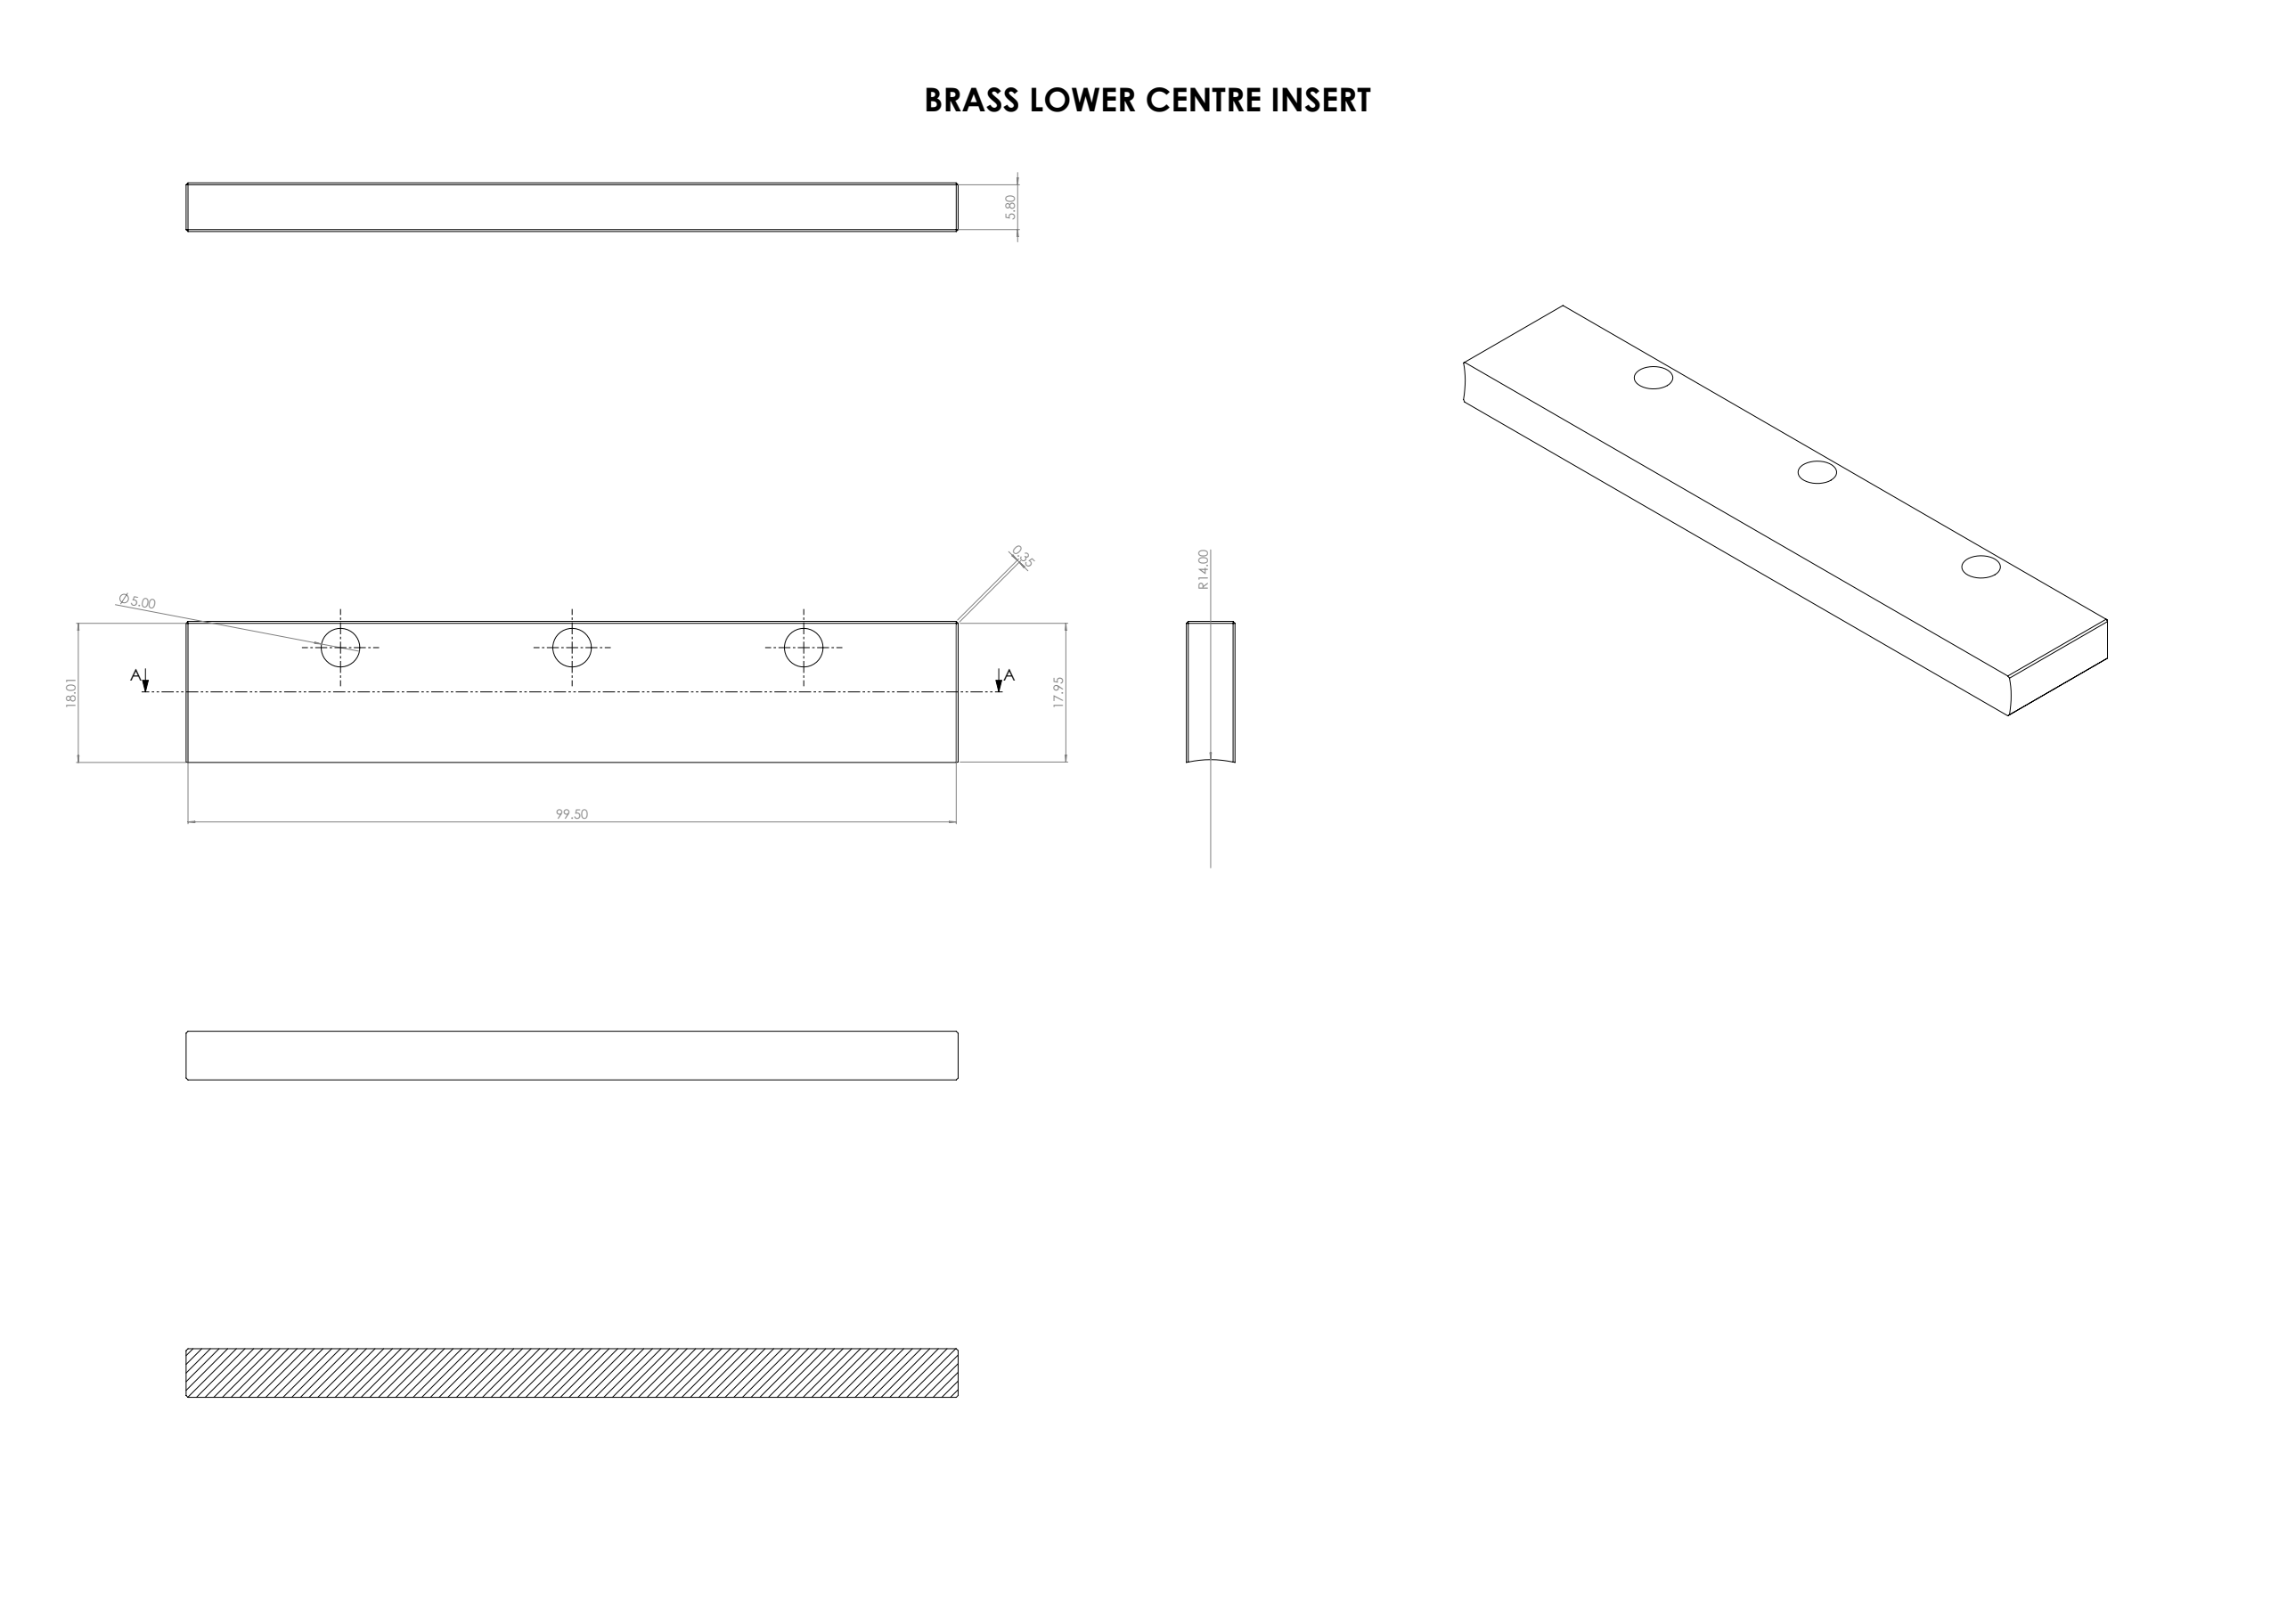
ISO-10303-21;
HEADER;
/* Generated by software containing ST-Developer
 * from STEP Tools, Inc. (www.steptools.com) 
 */

FILE_DESCRIPTION(
/* description */ (''),
/* implementation_level */ '2;1');

FILE_NAME(
/* name */ '02_Brass_Lower_Centre_Insert.step',
/* time_stamp */ '2026-10-21T01:59:45-07:00',
/* author */ (''),
/* organization */ (''),
/* preprocessor_version */ 'ST-DEVELOPER v20.2',
/* originating_system */ 'Autodesk Translation Framework v15.15.0.0',
/* authorisation */ '');

FILE_SCHEMA (('AUTOMOTIVE_DESIGN { 1 0 10303 214 3 1 1 }'));
ENDSEC;

DATA;
#10=MECHANICAL_DESIGN_GEOMETRIC_PRESENTATION_REPRESENTATION('',(#463),#18281);
#437=SHAPE_REPRESENTATION_RELATIONSHIP('SRR','None',#18339,#450);
#450=ADVANCED_BREP_SHAPE_REPRESENTATION('',(#481),#18268);
#463=STYLED_ITEM('',(#18467),#481);
#481=MANIFOLD_SOLID_BREP('Body1',#9085);
#494=CYLINDRICAL_SURFACE('',#9267,2.5);
#495=CYLINDRICAL_SURFACE('',#9269,2.5);
#496=CYLINDRICAL_SURFACE('',#9271,2.5);
#497=CYLINDRICAL_SURFACE('',#9273,14.);
#579=FACE_BOUND('',#1377,.T.);
#580=FACE_BOUND('',#1378,.T.);
#581=FACE_BOUND('',#1379,.T.);
#582=FACE_BOUND('',#1388,.T.);
#583=FACE_BOUND('',#1389,.T.);
#584=FACE_BOUND('',#1390,.T.);
#629=CIRCLE('',#9261,2.5);
#630=CIRCLE('',#9262,2.5);
#631=CIRCLE('',#9263,2.5);
#632=CIRCLE('',#9265,14.);
#633=CIRCLE('',#9268,2.5);
#634=CIRCLE('',#9270,2.5);
#635=CIRCLE('',#9272,2.5);
#636=CIRCLE('',#9274,14.);
#822=ELLIPSE('',#9249,19.7989898732233,14.);
#823=ELLIPSE('',#9254,19.7989898732235,14.);
#824=ELLIPSE('',#9256,19.7989898732233,14.);
#825=ELLIPSE('',#9259,19.7989898732235,14.);
#842=FACE_OUTER_BOUND('',#1364,.T.);
#843=FACE_OUTER_BOUND('',#1365,.T.);
#844=FACE_OUTER_BOUND('',#1366,.T.);
#845=FACE_OUTER_BOUND('',#1367,.T.);
#846=FACE_OUTER_BOUND('',#1368,.T.);
#847=FACE_OUTER_BOUND('',#1369,.T.);
#848=FACE_OUTER_BOUND('',#1370,.T.);
#849=FACE_OUTER_BOUND('',#1371,.T.);
#850=FACE_OUTER_BOUND('',#1372,.T.);
#851=FACE_OUTER_BOUND('',#1373,.T.);
#852=FACE_OUTER_BOUND('',#1374,.T.);
#853=FACE_OUTER_BOUND('',#1375,.T.);
#854=FACE_OUTER_BOUND('',#1376,.T.);
#855=FACE_OUTER_BOUND('',#1380,.T.);
#856=FACE_OUTER_BOUND('',#1381,.T.);
#857=FACE_OUTER_BOUND('',#1382,.T.);
#858=FACE_OUTER_BOUND('',#1383,.T.);
#859=FACE_OUTER_BOUND('',#1384,.T.);
#860=FACE_OUTER_BOUND('',#1385,.T.);
#861=FACE_OUTER_BOUND('',#1386,.T.);
#862=FACE_OUTER_BOUND('',#1387,.T.);
#1364=EDGE_LOOP('',(#5692,#5693,#5694));
#1365=EDGE_LOOP('',(#5695,#5696,#5697));
#1366=EDGE_LOOP('',(#5698,#5699,#5700));
#1367=EDGE_LOOP('',(#5701,#5702,#5703));
#1368=EDGE_LOOP('',(#5704,#5705,#5706,#5707));
#1369=EDGE_LOOP('',(#5708,#5709,#5710,#5711));
#1370=EDGE_LOOP('',(#5712,#5713,#5714,#5715));
#1371=EDGE_LOOP('',(#5716,#5717,#5718,#5719));
#1372=EDGE_LOOP('',(#5720,#5721,#5722,#5723));
#1373=EDGE_LOOP('',(#5724,#5725,#5726,#5727));
#1374=EDGE_LOOP('',(#5728,#5729,#5730,#5731));
#1375=EDGE_LOOP('',(#5732,#5733,#5734,#5735));
#1376=EDGE_LOOP('',(#5736,#5737,#5738,#5739));
#1377=EDGE_LOOP('',(#5740));
#1378=EDGE_LOOP('',(#5741));
#1379=EDGE_LOOP('',(#5742));
#1380=EDGE_LOOP('',(#5743,#5744,#5745,#5746));
#1381=EDGE_LOOP('',(#5747,#5748,#5749,#5750));
#1382=EDGE_LOOP('',(#5751,#5752,#5753,#5754));
#1383=EDGE_LOOP('',(#5755,#5756,#5757,#5758));
#1384=EDGE_LOOP('',(#5759,#5760,#5761,#5762));
#1385=EDGE_LOOP('',(#5763,#5764,#5765,#5766,#5767,#5768,#5769,#5770));
#1386=EDGE_LOOP('',(#5771,#5772,#5773,#5774));
#1387=EDGE_LOOP('',(#5775,#5776,#5777,#5778));
#1388=EDGE_LOOP('',(#5779));
#1389=EDGE_LOOP('',(#5780));
#1390=EDGE_LOOP('',(#5781));
#1936=LINE('',#12276,#2781);
#1937=LINE('',#12278,#2782);
#1938=LINE('',#12279,#2783);
#1939=LINE('',#12283,#2784);
#1940=LINE('',#12285,#2785);
#1941=LINE('',#12286,#2786);
#1942=LINE('',#12290,#2787);
#1943=LINE('',#12292,#2788);
#1944=LINE('',#12293,#2789);
#1945=LINE('',#12297,#2790);
#1946=LINE('',#12299,#2791);
#1947=LINE('',#12300,#2792);
#1948=LINE('',#12305,#2793);
#1949=LINE('',#12306,#2794);
#1950=LINE('',#12308,#2795);
#1951=LINE('',#12309,#2796);
#1952=LINE('',#12311,#2797);
#1953=LINE('',#12312,#2798);
#1954=LINE('',#12314,#2799);
#1955=LINE('',#12315,#2800);
#1956=LINE('',#12320,#2801);
#1957=LINE('',#12321,#2802);
#1958=LINE('',#12326,#2803);
#1959=LINE('',#12327,#2804);
#1960=LINE('',#12329,#2805);
#1961=LINE('',#12330,#2806);
#1962=LINE('',#12335,#2807);
#1963=LINE('',#12336,#2808);
#1964=LINE('',#12338,#2809);
#1965=LINE('',#12351,#2810);
#1966=LINE('',#12355,#2811);
#1967=LINE('',#12359,#2812);
#1968=LINE('',#12361,#2813);
#2781=VECTOR('',#9976,10.);
#2782=VECTOR('',#9977,10.);
#2783=VECTOR('',#9978,10.);
#2784=VECTOR('',#9981,10.);
#2785=VECTOR('',#9982,10.);
#2786=VECTOR('',#9983,10.);
#2787=VECTOR('',#9986,10.);
#2788=VECTOR('',#9987,10.);
#2789=VECTOR('',#9988,10.);
#2790=VECTOR('',#9991,10.);
#2791=VECTOR('',#9992,10.);
#2792=VECTOR('',#9993,10.);
#2793=VECTOR('',#9998,10.);
#2794=VECTOR('',#9999,10.);
#2795=VECTOR('',#10002,10.);
#2796=VECTOR('',#10003,10.);
#2797=VECTOR('',#10006,10.);
#2798=VECTOR('',#10007,10.);
#2799=VECTOR('',#10010,10.);
#2800=VECTOR('',#10011,10.);
#2801=VECTOR('',#10016,10.);
#2802=VECTOR('',#10017,10.);
#2803=VECTOR('',#10022,10.);
#2804=VECTOR('',#10023,10.);
#2805=VECTOR('',#10026,10.);
#2806=VECTOR('',#10027,10.);
#2807=VECTOR('',#10032,10.);
#2808=VECTOR('',#10033,10.);
#2809=VECTOR('',#10036,10.);
#2810=VECTOR('',#10053,2.5);
#2811=VECTOR('',#10058,2.5);
#2812=VECTOR('',#10063,2.5);
#2813=VECTOR('',#10066,10.);
#3626=VERTEX_POINT('',#12274);
#3627=VERTEX_POINT('',#12275);
#3628=VERTEX_POINT('',#12277);
#3629=VERTEX_POINT('',#12281);
#3630=VERTEX_POINT('',#12282);
#3631=VERTEX_POINT('',#12284);
#3632=VERTEX_POINT('',#12288);
#3633=VERTEX_POINT('',#12289);
#3634=VERTEX_POINT('',#12291);
#3635=VERTEX_POINT('',#12295);
#3636=VERTEX_POINT('',#12296);
#3637=VERTEX_POINT('',#12298);
#3638=VERTEX_POINT('',#12302);
#3639=VERTEX_POINT('',#12303);
#3640=VERTEX_POINT('',#12317);
#3641=VERTEX_POINT('',#12318);
#3642=VERTEX_POINT('',#12323);
#3643=VERTEX_POINT('',#12324);
#3644=VERTEX_POINT('',#12332);
#3645=VERTEX_POINT('',#12333);
#3646=VERTEX_POINT('',#12339);
#3647=VERTEX_POINT('',#12341);
#3648=VERTEX_POINT('',#12343);
#3649=VERTEX_POINT('',#12349);
#3650=VERTEX_POINT('',#12353);
#3651=VERTEX_POINT('',#12357);
#4418=EDGE_CURVE('',#3626,#3627,#1936,.T.);
#4419=EDGE_CURVE('',#3628,#3626,#1937,.T.);
#4420=EDGE_CURVE('',#3627,#3628,#1938,.T.);
#4421=EDGE_CURVE('',#3629,#3630,#1939,.T.);
#4422=EDGE_CURVE('',#3631,#3629,#1940,.T.);
#4423=EDGE_CURVE('',#3630,#3631,#1941,.T.);
#4424=EDGE_CURVE('',#3632,#3633,#1942,.T.);
#4425=EDGE_CURVE('',#3634,#3632,#1943,.T.);
#4426=EDGE_CURVE('',#3633,#3634,#1944,.T.);
#4427=EDGE_CURVE('',#3635,#3636,#1945,.T.);
#4428=EDGE_CURVE('',#3637,#3635,#1946,.T.);
#4429=EDGE_CURVE('',#3636,#3637,#1947,.T.);
#4430=EDGE_CURVE('',#3638,#3639,#822,.T.);
#4431=EDGE_CURVE('',#3639,#3637,#1948,.T.);
#4432=EDGE_CURVE('',#3635,#3638,#1949,.T.);
#4433=EDGE_CURVE('',#3629,#3636,#1950,.T.);
#4434=EDGE_CURVE('',#3637,#3631,#1951,.T.);
#4435=EDGE_CURVE('',#3632,#3635,#1952,.T.);
#4436=EDGE_CURVE('',#3636,#3634,#1953,.T.);
#4437=EDGE_CURVE('',#3627,#3633,#1954,.T.);
#4438=EDGE_CURVE('',#3634,#3626,#1955,.T.);
#4439=EDGE_CURVE('',#3640,#3641,#823,.T.);
#4440=EDGE_CURVE('',#3641,#3632,#1956,.T.);
#4441=EDGE_CURVE('',#3633,#3640,#1957,.T.);
#4442=EDGE_CURVE('',#3642,#3643,#824,.T.);
#4443=EDGE_CURVE('',#3643,#3630,#1958,.T.);
#4444=EDGE_CURVE('',#3631,#3642,#1959,.T.);
#4445=EDGE_CURVE('',#3626,#3629,#1960,.T.);
#4446=EDGE_CURVE('',#3630,#3628,#1961,.T.);
#4447=EDGE_CURVE('',#3644,#3645,#825,.T.);
#4448=EDGE_CURVE('',#3645,#3627,#1962,.T.);
#4449=EDGE_CURVE('',#3628,#3644,#1963,.T.);
#4450=EDGE_CURVE('',#3641,#3638,#1964,.T.);
#4451=EDGE_CURVE('',#3646,#3646,#629,.T.);
#4452=EDGE_CURVE('',#3647,#3647,#630,.T.);
#4453=EDGE_CURVE('',#3648,#3648,#631,.T.);
#4454=EDGE_CURVE('',#3645,#3640,#632,.T.);
#4455=EDGE_CURVE('',#3649,#3649,#633,.T.);
#4456=EDGE_CURVE('',#3649,#3648,#1965,.T.);
#4457=EDGE_CURVE('',#3650,#3650,#634,.T.);
#4458=EDGE_CURVE('',#3650,#3647,#1966,.T.);
#4459=EDGE_CURVE('',#3651,#3651,#635,.T.);
#4460=EDGE_CURVE('',#3651,#3646,#1967,.T.);
#4461=EDGE_CURVE('',#3643,#3644,#1968,.T.);
#4462=EDGE_CURVE('',#3639,#3642,#636,.T.);
#5692=ORIENTED_EDGE('',*,*,#4418,.F.);
#5693=ORIENTED_EDGE('',*,*,#4419,.F.);
#5694=ORIENTED_EDGE('',*,*,#4420,.F.);
#5695=ORIENTED_EDGE('',*,*,#4421,.F.);
#5696=ORIENTED_EDGE('',*,*,#4422,.F.);
#5697=ORIENTED_EDGE('',*,*,#4423,.F.);
#5698=ORIENTED_EDGE('',*,*,#4424,.F.);
#5699=ORIENTED_EDGE('',*,*,#4425,.F.);
#5700=ORIENTED_EDGE('',*,*,#4426,.F.);
#5701=ORIENTED_EDGE('',*,*,#4427,.F.);
#5702=ORIENTED_EDGE('',*,*,#4428,.F.);
#5703=ORIENTED_EDGE('',*,*,#4429,.F.);
#5704=ORIENTED_EDGE('',*,*,#4430,.T.);
#5705=ORIENTED_EDGE('',*,*,#4431,.T.);
#5706=ORIENTED_EDGE('',*,*,#4428,.T.);
#5707=ORIENTED_EDGE('',*,*,#4432,.T.);
#5708=ORIENTED_EDGE('',*,*,#4422,.T.);
#5709=ORIENTED_EDGE('',*,*,#4433,.T.);
#5710=ORIENTED_EDGE('',*,*,#4429,.T.);
#5711=ORIENTED_EDGE('',*,*,#4434,.T.);
#5712=ORIENTED_EDGE('',*,*,#4425,.T.);
#5713=ORIENTED_EDGE('',*,*,#4435,.T.);
#5714=ORIENTED_EDGE('',*,*,#4427,.T.);
#5715=ORIENTED_EDGE('',*,*,#4436,.T.);
#5716=ORIENTED_EDGE('',*,*,#4418,.T.);
#5717=ORIENTED_EDGE('',*,*,#4437,.T.);
#5718=ORIENTED_EDGE('',*,*,#4426,.T.);
#5719=ORIENTED_EDGE('',*,*,#4438,.T.);
#5720=ORIENTED_EDGE('',*,*,#4439,.T.);
#5721=ORIENTED_EDGE('',*,*,#4440,.T.);
#5722=ORIENTED_EDGE('',*,*,#4424,.T.);
#5723=ORIENTED_EDGE('',*,*,#4441,.T.);
#5724=ORIENTED_EDGE('',*,*,#4442,.T.);
#5725=ORIENTED_EDGE('',*,*,#4443,.T.);
#5726=ORIENTED_EDGE('',*,*,#4423,.T.);
#5727=ORIENTED_EDGE('',*,*,#4444,.T.);
#5728=ORIENTED_EDGE('',*,*,#4419,.T.);
#5729=ORIENTED_EDGE('',*,*,#4445,.T.);
#5730=ORIENTED_EDGE('',*,*,#4421,.T.);
#5731=ORIENTED_EDGE('',*,*,#4446,.T.);
#5732=ORIENTED_EDGE('',*,*,#4447,.T.);
#5733=ORIENTED_EDGE('',*,*,#4448,.T.);
#5734=ORIENTED_EDGE('',*,*,#4420,.T.);
#5735=ORIENTED_EDGE('',*,*,#4449,.T.);
#5736=ORIENTED_EDGE('',*,*,#4432,.F.);
#5737=ORIENTED_EDGE('',*,*,#4435,.F.);
#5738=ORIENTED_EDGE('',*,*,#4440,.F.);
#5739=ORIENTED_EDGE('',*,*,#4450,.T.);
#5740=ORIENTED_EDGE('',*,*,#4451,.T.);
#5741=ORIENTED_EDGE('',*,*,#4452,.T.);
#5742=ORIENTED_EDGE('',*,*,#4453,.T.);
#5743=ORIENTED_EDGE('',*,*,#4441,.F.);
#5744=ORIENTED_EDGE('',*,*,#4437,.F.);
#5745=ORIENTED_EDGE('',*,*,#4448,.F.);
#5746=ORIENTED_EDGE('',*,*,#4454,.T.);
#5747=ORIENTED_EDGE('',*,*,#4433,.F.);
#5748=ORIENTED_EDGE('',*,*,#4445,.F.);
#5749=ORIENTED_EDGE('',*,*,#4438,.F.);
#5750=ORIENTED_EDGE('',*,*,#4436,.F.);
#5751=ORIENTED_EDGE('',*,*,#4455,.F.);
#5752=ORIENTED_EDGE('',*,*,#4456,.T.);
#5753=ORIENTED_EDGE('',*,*,#4453,.F.);
#5754=ORIENTED_EDGE('',*,*,#4456,.F.);
#5755=ORIENTED_EDGE('',*,*,#4457,.F.);
#5756=ORIENTED_EDGE('',*,*,#4458,.T.);
#5757=ORIENTED_EDGE('',*,*,#4452,.F.);
#5758=ORIENTED_EDGE('',*,*,#4458,.F.);
#5759=ORIENTED_EDGE('',*,*,#4459,.F.);
#5760=ORIENTED_EDGE('',*,*,#4460,.T.);
#5761=ORIENTED_EDGE('',*,*,#4451,.F.);
#5762=ORIENTED_EDGE('',*,*,#4460,.F.);
#5763=ORIENTED_EDGE('',*,*,#4430,.F.);
#5764=ORIENTED_EDGE('',*,*,#4450,.F.);
#5765=ORIENTED_EDGE('',*,*,#4439,.F.);
#5766=ORIENTED_EDGE('',*,*,#4454,.F.);
#5767=ORIENTED_EDGE('',*,*,#4447,.F.);
#5768=ORIENTED_EDGE('',*,*,#4461,.F.);
#5769=ORIENTED_EDGE('',*,*,#4442,.F.);
#5770=ORIENTED_EDGE('',*,*,#4462,.F.);
#5771=ORIENTED_EDGE('',*,*,#4431,.F.);
#5772=ORIENTED_EDGE('',*,*,#4462,.T.);
#5773=ORIENTED_EDGE('',*,*,#4444,.F.);
#5774=ORIENTED_EDGE('',*,*,#4434,.F.);
#5775=ORIENTED_EDGE('',*,*,#4443,.F.);
#5776=ORIENTED_EDGE('',*,*,#4461,.T.);
#5777=ORIENTED_EDGE('',*,*,#4449,.F.);
#5778=ORIENTED_EDGE('',*,*,#4446,.F.);
#5779=ORIENTED_EDGE('',*,*,#4455,.T.);
#5780=ORIENTED_EDGE('',*,*,#4457,.T.);
#5781=ORIENTED_EDGE('',*,*,#4459,.T.);
#8240=PLANE('',#9244);
#8241=PLANE('',#9245);
#8242=PLANE('',#9246);
#8243=PLANE('',#9247);
#8244=PLANE('',#9248);
#8245=PLANE('',#9250);
#8246=PLANE('',#9251);
#8247=PLANE('',#9252);
#8248=PLANE('',#9253);
#8249=PLANE('',#9255);
#8250=PLANE('',#9257);
#8251=PLANE('',#9258);
#8252=PLANE('',#9260);
#8253=PLANE('',#9264);
#8254=PLANE('',#9266);
#8255=PLANE('',#9275);
#8256=PLANE('',#9276);
#8563=ADVANCED_FACE('',(#842),#8240,.T.);
#8564=ADVANCED_FACE('',(#843),#8241,.T.);
#8565=ADVANCED_FACE('',(#844),#8242,.T.);
#8566=ADVANCED_FACE('',(#845),#8243,.T.);
#8567=ADVANCED_FACE('',(#846),#8244,.T.);
#8568=ADVANCED_FACE('',(#847),#8245,.T.);
#8569=ADVANCED_FACE('',(#848),#8246,.T.);
#8570=ADVANCED_FACE('',(#849),#8247,.T.);
#8571=ADVANCED_FACE('',(#850),#8248,.T.);
#8572=ADVANCED_FACE('',(#851),#8249,.T.);
#8573=ADVANCED_FACE('',(#852),#8250,.T.);
#8574=ADVANCED_FACE('',(#853),#8251,.T.);
#8575=ADVANCED_FACE('',(#854,#579,#580,#581),#8252,.T.);
#8576=ADVANCED_FACE('',(#855),#8253,.T.);
#8577=ADVANCED_FACE('',(#856),#8254,.T.);
#8578=ADVANCED_FACE('',(#857),#494,.F.);
#8579=ADVANCED_FACE('',(#858),#495,.F.);
#8580=ADVANCED_FACE('',(#859),#496,.F.);
#8581=ADVANCED_FACE('',(#860),#497,.F.);
#8582=ADVANCED_FACE('',(#861),#8255,.F.);
#8583=ADVANCED_FACE('',(#862,#582,#583,#584),#8256,.T.);
#9085=CLOSED_SHELL('',(#8563,#8564,#8565,#8566,#8567,#8568,#8569,#8570,
#8571,#8572,#8573,#8574,#8575,#8576,#8577,#8578,#8579,#8580,#8581,#8582,
#8583));
#9243=AXIS2_PLACEMENT_3D('',#12272,#9972,#9973);
#9244=AXIS2_PLACEMENT_3D('',#12273,#9974,#9975);
#9245=AXIS2_PLACEMENT_3D('',#12280,#9979,#9980);
#9246=AXIS2_PLACEMENT_3D('',#12287,#9984,#9985);
#9247=AXIS2_PLACEMENT_3D('',#12294,#9989,#9990);
#9248=AXIS2_PLACEMENT_3D('',#12301,#9994,#9995);
#9249=AXIS2_PLACEMENT_3D('',#12304,#9996,#9997);
#9250=AXIS2_PLACEMENT_3D('',#12307,#10000,#10001);
#9251=AXIS2_PLACEMENT_3D('',#12310,#10004,#10005);
#9252=AXIS2_PLACEMENT_3D('',#12313,#10008,#10009);
#9253=AXIS2_PLACEMENT_3D('',#12316,#10012,#10013);
#9254=AXIS2_PLACEMENT_3D('',#12319,#10014,#10015);
#9255=AXIS2_PLACEMENT_3D('',#12322,#10018,#10019);
#9256=AXIS2_PLACEMENT_3D('',#12325,#10020,#10021);
#9257=AXIS2_PLACEMENT_3D('',#12328,#10024,#10025);
#9258=AXIS2_PLACEMENT_3D('',#12331,#10028,#10029);
#9259=AXIS2_PLACEMENT_3D('',#12334,#10030,#10031);
#9260=AXIS2_PLACEMENT_3D('',#12337,#10034,#10035);
#9261=AXIS2_PLACEMENT_3D('',#12340,#10037,#10038);
#9262=AXIS2_PLACEMENT_3D('',#12342,#10039,#10040);
#9263=AXIS2_PLACEMENT_3D('',#12344,#10041,#10042);
#9264=AXIS2_PLACEMENT_3D('',#12345,#10043,#10044);
#9265=AXIS2_PLACEMENT_3D('',#12346,#10045,#10046);
#9266=AXIS2_PLACEMENT_3D('',#12347,#10047,#10048);
#9267=AXIS2_PLACEMENT_3D('',#12348,#10049,#10050);
#9268=AXIS2_PLACEMENT_3D('',#12350,#10051,#10052);
#9269=AXIS2_PLACEMENT_3D('',#12352,#10054,#10055);
#9270=AXIS2_PLACEMENT_3D('',#12354,#10056,#10057);
#9271=AXIS2_PLACEMENT_3D('',#12356,#10059,#10060);
#9272=AXIS2_PLACEMENT_3D('',#12358,#10061,#10062);
#9273=AXIS2_PLACEMENT_3D('',#12360,#10064,#10065);
#9274=AXIS2_PLACEMENT_3D('',#12362,#10067,#10068);
#9275=AXIS2_PLACEMENT_3D('',#12363,#10069,#10070);
#9276=AXIS2_PLACEMENT_3D('',#12364,#10071,#10072);
#9972=DIRECTION('axis',(0.,0.,1.));
#9973=DIRECTION('refdir',(1.,0.,0.));
#9974=DIRECTION('center_axis',(0.57735026918962,0.577350269189628,-0.57735026918963));
#9975=DIRECTION('ref_axis',(-0.707106781186554,0.,-0.707106781186541));
#9976=DIRECTION('',(0.707106781186554,0.,0.707106781186541));
#9977=DIRECTION('',(0.,-0.707106781186549,-0.707106781186546));
#9978=DIRECTION('',(-0.707106781186552,0.707106781186543,0.));
#9979=DIRECTION('center_axis',(-0.577350269189622,0.577350269189627,-0.577350269189629));
#9980=DIRECTION('ref_axis',(-0.707106781186552,0.,0.707106781186543));
#9981=DIRECTION('',(0.,0.707106781186549,0.707106781186546));
#9982=DIRECTION('',(0.707106781186552,0.,-0.707106781186543));
#9983=DIRECTION('',(-0.707106781186547,-0.707106781186548,-6.2803698347351E-15));
#9984=DIRECTION('center_axis',(0.57735026918962,-0.577350269189628,-0.57735026918963));
#9985=DIRECTION('ref_axis',(-0.707106781186554,0.,-0.707106781186541));
#9986=DIRECTION('',(0.707106781186552,0.707106781186543,0.));
#9987=DIRECTION('',(0.,-0.707106781186549,0.707106781186546));
#9988=DIRECTION('',(-0.707106781186554,0.,-0.707106781186541));
#9989=DIRECTION('center_axis',(-0.577350269189622,-0.577350269189627,-0.577350269189629));
#9990=DIRECTION('ref_axis',(-0.707106781186552,0.,0.707106781186543));
#9991=DIRECTION('',(0.,0.707106781186549,-0.707106781186546));
#9992=DIRECTION('',(0.707106781186547,-0.707106781186548,6.2803698347351E-15));
#9993=DIRECTION('',(-0.707106781186552,0.,0.707106781186543));
#9994=DIRECTION('center_axis',(-0.707106781186548,-0.707106781186547,0.));
#9995=DIRECTION('ref_axis',(0.,0.,1.));
#9996=DIRECTION('center_axis',(0.707106781186548,0.707106781186547,0.));
#9997=DIRECTION('ref_axis',(-0.707106781186547,0.707106781186548,0.));
#9998=DIRECTION('',(0.,0.,-1.));
#9999=DIRECTION('',(0.,0.,1.));
#10000=DIRECTION('center_axis',(-0.707106781186543,0.,-0.707106781186552));
#10001=DIRECTION('ref_axis',(-0.707106781186552,0.,0.707106781186543));
#10002=DIRECTION('',(0.,-1.,0.));
#10003=DIRECTION('',(0.,1.,0.));
#10004=DIRECTION('center_axis',(0.,-0.707106781186546,-0.707106781186549));
#10005=DIRECTION('ref_axis',(-1.,0.,0.));
#10006=DIRECTION('',(-1.,0.,0.));
#10007=DIRECTION('',(1.,0.,0.));
#10008=DIRECTION('center_axis',(0.707106781186541,0.,-0.707106781186554));
#10009=DIRECTION('ref_axis',(-0.707106781186554,0.,-0.707106781186541));
#10010=DIRECTION('',(0.,-1.,0.));
#10011=DIRECTION('',(0.,1.,0.));
#10012=DIRECTION('center_axis',(0.707106781186543,-0.707106781186552,0.));
#10013=DIRECTION('ref_axis',(0.,0.,-1.));
#10014=DIRECTION('center_axis',(-0.707106781186543,0.707106781186552,0.));
#10015=DIRECTION('ref_axis',(0.707106781186552,0.707106781186543,0.));
#10016=DIRECTION('',(0.,0.,-1.));
#10017=DIRECTION('',(0.,0.,1.));
#10018=DIRECTION('center_axis',(-0.707106781186548,0.707106781186547,0.));
#10019=DIRECTION('ref_axis',(0.,0.,1.));
#10020=DIRECTION('center_axis',(0.707106781186548,-0.707106781186547,0.));
#10021=DIRECTION('ref_axis',(0.707106781186547,0.707106781186548,0.));
#10022=DIRECTION('',(0.,0.,-1.));
#10023=DIRECTION('',(0.,0.,1.));
#10024=DIRECTION('center_axis',(0.,0.707106781186546,-0.707106781186549));
#10025=DIRECTION('ref_axis',(-1.,0.,0.));
#10026=DIRECTION('',(-1.,0.,0.));
#10027=DIRECTION('',(1.,0.,0.));
#10028=DIRECTION('center_axis',(0.707106781186543,0.707106781186552,0.));
#10029=DIRECTION('ref_axis',(0.,0.,-1.));
#10030=DIRECTION('center_axis',(-0.707106781186543,-0.707106781186552,0.));
#10031=DIRECTION('ref_axis',(-0.707106781186552,0.707106781186543,0.));
#10032=DIRECTION('',(0.,0.,-1.));
#10033=DIRECTION('',(0.,0.,1.));
#10034=DIRECTION('center_axis',(0.,-1.,0.));
#10035=DIRECTION('ref_axis',(0.,0.,-1.));
#10036=DIRECTION('',(-1.,0.,0.));
#10037=DIRECTION('center_axis',(0.,1.,0.));
#10038=DIRECTION('ref_axis',(1.,0.,0.));
#10039=DIRECTION('center_axis',(0.,1.,0.));
#10040=DIRECTION('ref_axis',(1.,0.,0.));
#10041=DIRECTION('center_axis',(0.,1.,0.));
#10042=DIRECTION('ref_axis',(1.,0.,0.));
#10043=DIRECTION('center_axis',(1.,0.,0.));
#10044=DIRECTION('ref_axis',(0.,0.,-1.));
#10045=DIRECTION('center_axis',(-1.,0.,0.));
#10046=DIRECTION('ref_axis',(0.,0.,-1.));
#10047=DIRECTION('center_axis',(0.,0.,-1.));
#10048=DIRECTION('ref_axis',(0.,1.,0.));
#10049=DIRECTION('center_axis',(0.,-1.,0.));
#10050=DIRECTION('ref_axis',(1.,0.,0.));
#10051=DIRECTION('center_axis',(0.,-1.,0.));
#10052=DIRECTION('ref_axis',(1.,0.,0.));
#10053=DIRECTION('',(0.,-1.,0.));
#10054=DIRECTION('center_axis',(0.,-1.,0.));
#10055=DIRECTION('ref_axis',(1.,0.,0.));
#10056=DIRECTION('center_axis',(0.,-1.,0.));
#10057=DIRECTION('ref_axis',(1.,0.,0.));
#10058=DIRECTION('',(0.,-1.,0.));
#10059=DIRECTION('center_axis',(0.,-1.,0.));
#10060=DIRECTION('ref_axis',(1.,0.,0.));
#10061=DIRECTION('center_axis',(0.,-1.,0.));
#10062=DIRECTION('ref_axis',(1.,0.,0.));
#10063=DIRECTION('',(0.,-1.,0.));
#10064=DIRECTION('center_axis',(1.,0.,0.));
#10065=DIRECTION('ref_axis',(0.,0.,-1.));
#10066=DIRECTION('',(1.,0.,0.));
#10067=DIRECTION('center_axis',(1.,0.,0.));
#10068=DIRECTION('ref_axis',(0.,0.,-1.));
#10069=DIRECTION('center_axis',(1.,0.,0.));
#10070=DIRECTION('ref_axis',(0.,0.,-1.));
#10071=DIRECTION('center_axis',(0.,1.,0.));
#10072=DIRECTION('ref_axis',(0.,0.,1.));
#12272=CARTESIAN_POINT('',(0.,0.,0.));
#12273=CARTESIAN_POINT('Origin',(99.75,3.15,15.85));
#12274=CARTESIAN_POINT('',(99.75,2.9,15.6));
#12275=CARTESIAN_POINT('',(100.,2.9,15.85));
#12276=CARTESIAN_POINT('',(99.75,2.9,15.6));
#12277=CARTESIAN_POINT('',(99.75,3.15,15.85));
#12278=CARTESIAN_POINT('',(99.75,3.15,15.85));
#12279=CARTESIAN_POINT('',(100.,2.9,15.85));
#12280=CARTESIAN_POINT('Origin',(0.,2.9,15.85));
#12281=CARTESIAN_POINT('',(0.25,2.9,15.6));
#12282=CARTESIAN_POINT('',(0.25,3.15,15.85));
#12283=CARTESIAN_POINT('',(0.25,2.9,15.6));
#12284=CARTESIAN_POINT('',(0.,2.9,15.85));
#12285=CARTESIAN_POINT('',(0.,2.9,15.85));
#12286=CARTESIAN_POINT('',(0.25,3.15,15.85));
#12287=CARTESIAN_POINT('Origin',(99.75,-2.9,15.6));
#12288=CARTESIAN_POINT('',(99.75,-3.15,15.85));
#12289=CARTESIAN_POINT('',(100.,-2.9,15.85));
#12290=CARTESIAN_POINT('',(99.75,-3.15,15.85));
#12291=CARTESIAN_POINT('',(99.75,-2.9,15.6));
#12292=CARTESIAN_POINT('',(99.75,-2.9,15.6));
#12293=CARTESIAN_POINT('',(100.,-2.9,15.85));
#12294=CARTESIAN_POINT('Origin',(0.,-2.9,15.85));
#12295=CARTESIAN_POINT('',(0.25,-3.15,15.85));
#12296=CARTESIAN_POINT('',(0.25,-2.9,15.6));
#12297=CARTESIAN_POINT('',(0.25,-3.15,15.85));
#12298=CARTESIAN_POINT('',(0.,-2.9,15.85));
#12299=CARTESIAN_POINT('',(0.,-2.9,15.85));
#12300=CARTESIAN_POINT('',(0.25,-2.9,15.6));
#12301=CARTESIAN_POINT('Origin',(0.125,-3.025,31.275));
#12302=CARTESIAN_POINT('',(0.25,-3.15,33.8589773110664));
#12303=CARTESIAN_POINT('',(0.,-2.9,33.8036501212914));
#12304=CARTESIAN_POINT('Origin',(-2.9,0.,47.5));
#12305=CARTESIAN_POINT('',(0.,-2.9,31.275));
#12306=CARTESIAN_POINT('',(0.25,-3.15,31.275));
#12307=CARTESIAN_POINT('Origin',(0.125,-1.575,15.725));
#12308=CARTESIAN_POINT('',(0.25,-1.575,15.6));
#12309=CARTESIAN_POINT('',(0.,-1.575,15.85));
#12310=CARTESIAN_POINT('Origin',(0.,-3.025,15.725));
#12311=CARTESIAN_POINT('',(0.,-3.15,15.85));
#12312=CARTESIAN_POINT('',(0.,-2.9,15.6));
#12313=CARTESIAN_POINT('Origin',(99.875,-1.575,15.725));
#12314=CARTESIAN_POINT('',(100.,-1.575,15.85));
#12315=CARTESIAN_POINT('',(99.75,-1.575,15.6));
#12316=CARTESIAN_POINT('Origin',(99.875,-3.025,31.275));
#12317=CARTESIAN_POINT('',(100.,-2.9,33.8036501212914));
#12318=CARTESIAN_POINT('',(99.75,-3.15,33.8589773110664));
#12319=CARTESIAN_POINT('Origin',(102.9,0.,47.5));
#12320=CARTESIAN_POINT('',(99.75,-3.15,31.275));
#12321=CARTESIAN_POINT('',(100.,-2.9,31.275));
#12322=CARTESIAN_POINT('Origin',(0.125,3.025,20.825));
#12323=CARTESIAN_POINT('',(0.,2.9,33.8036501212914));
#12324=CARTESIAN_POINT('',(0.25,3.15,33.8589773110664));
#12325=CARTESIAN_POINT('Origin',(-2.9,0.,47.5));
#12326=CARTESIAN_POINT('',(0.25,3.15,20.825));
#12327=CARTESIAN_POINT('',(0.,2.9,20.825));
#12328=CARTESIAN_POINT('Origin',(0.,3.025,15.725));
#12329=CARTESIAN_POINT('',(0.,2.9,15.6));
#12330=CARTESIAN_POINT('',(0.,3.15,15.85));
#12331=CARTESIAN_POINT('Origin',(99.875,3.025,20.825));
#12332=CARTESIAN_POINT('',(99.75,3.15,33.8589773110664));
#12333=CARTESIAN_POINT('',(100.,2.9,33.8036501212914));
#12334=CARTESIAN_POINT('Origin',(102.9,0.,47.5));
#12335=CARTESIAN_POINT('',(100.,2.9,20.825));
#12336=CARTESIAN_POINT('',(99.75,3.15,20.825));
#12337=CARTESIAN_POINT('Origin',(0.,-3.15,36.5));
#12338=CARTESIAN_POINT('',(0.,-3.15,33.8589773110664));
#12339=CARTESIAN_POINT('',(77.5,-3.15,19.));
#12340=CARTESIAN_POINT('Origin',(80.,-3.15,19.));
#12341=CARTESIAN_POINT('',(47.5,-3.15,19.));
#12342=CARTESIAN_POINT('Origin',(50.,-3.15,19.));
#12343=CARTESIAN_POINT('',(17.5,-3.15,19.));
#12344=CARTESIAN_POINT('Origin',(20.,-3.15,19.));
#12345=CARTESIAN_POINT('Origin',(100.,0.,26.05));
#12346=CARTESIAN_POINT('Origin',(100.,0.,47.5));
#12347=CARTESIAN_POINT('Origin',(0.,-3.15,15.6));
#12348=CARTESIAN_POINT('Origin',(20.,3.15,19.));
#12349=CARTESIAN_POINT('',(17.5,3.15,19.));
#12350=CARTESIAN_POINT('Origin',(20.,3.15,19.));
#12351=CARTESIAN_POINT('',(17.5,3.15,19.));
#12352=CARTESIAN_POINT('Origin',(50.,3.15,19.));
#12353=CARTESIAN_POINT('',(47.5,3.15,19.));
#12354=CARTESIAN_POINT('Origin',(50.,3.15,19.));
#12355=CARTESIAN_POINT('',(47.5,3.15,19.));
#12356=CARTESIAN_POINT('Origin',(80.,3.15,19.));
#12357=CARTESIAN_POINT('',(77.5,3.15,19.));
#12358=CARTESIAN_POINT('Origin',(80.,3.15,19.));
#12359=CARTESIAN_POINT('',(77.5,3.15,19.));
#12360=CARTESIAN_POINT('Origin',(0.,0.,47.5));
#12361=CARTESIAN_POINT('',(0.,3.15,33.8589773110664));
#12362=CARTESIAN_POINT('Origin',(0.,0.,47.5));
#12363=CARTESIAN_POINT('Origin',(0.,0.,26.05));
#12364=CARTESIAN_POINT('Origin',(0.,3.15,15.6));
#18253=UNCERTAINTY_MEASURE_WITH_UNIT(LENGTH_MEASURE(0.01),#18282,
'DISTANCE_ACCURACY_VALUE',
'Maximum model space distance between geometric entities at asserted c
onnectivities');
#18266=UNCERTAINTY_MEASURE_WITH_UNIT(LENGTH_MEASURE(0.01),#18282,
'DISTANCE_ACCURACY_VALUE',
'Maximum model space distance between geometric entities at asserted c
onnectivities');
#18268=(
GEOMETRIC_REPRESENTATION_CONTEXT(3)
GLOBAL_UNCERTAINTY_ASSIGNED_CONTEXT((#18253))
GLOBAL_UNIT_ASSIGNED_CONTEXT((#18282,#18284,#18285))
REPRESENTATION_CONTEXT('','3D')
);
#18281=(
GEOMETRIC_REPRESENTATION_CONTEXT(3)
GLOBAL_UNCERTAINTY_ASSIGNED_CONTEXT((#18266))
GLOBAL_UNIT_ASSIGNED_CONTEXT((#18282,#18284,#18285))
REPRESENTATION_CONTEXT('','3D')
);
#18282=(
LENGTH_UNIT()
NAMED_UNIT(*)
SI_UNIT(.MILLI.,.METRE.)
);
#18284=(
NAMED_UNIT(*)
PLANE_ANGLE_UNIT()
SI_UNIT($,.RADIAN.)
);
#18285=(
NAMED_UNIT(*)
SI_UNIT($,.STERADIAN.)
SOLID_ANGLE_UNIT()
);
#18287=SHAPE_DEFINITION_REPRESENTATION(#18301,#18339);
#18301=PRODUCT_DEFINITION_SHAPE('',$,#18354);
#18339=SHAPE_REPRESENTATION('',(#9243),#18268);
#18352=PRODUCT_DEFINITION_CONTEXT('part definition',#18396,'design');
#18354=PRODUCT_DEFINITION('2026-10-20-13-03-17-896',
'02_Brass_Lower_Centre_Insert',#18368,#18352);
#18368=PRODUCT_DEFINITION_FORMATION('',$,#18399);
#18396=APPLICATION_CONTEXT(
'Core Data for Automotive Mechanical Design Process');
#18397=PRODUCT_CONTEXT('part definition',#18396,'mechanical');
#18399=PRODUCT('2026-10-20-13-03-17-896','02_Brass_Lower_Centre_Insert',
$,(#18397));
#18461=COLOUR_RGB('Sky Blue',0.24,0.69,0.87);
#18462=FILL_AREA_STYLE_COLOUR('',#18461);
#18463=FILL_AREA_STYLE('',(#18462));
#18464=SURFACE_STYLE_FILL_AREA(#18463);
#18465=SURFACE_SIDE_STYLE('',(#18464));
#18466=SURFACE_STYLE_USAGE(.BOTH.,#18465);
#18467=PRESENTATION_STYLE_ASSIGNMENT((#18466));
ENDSEC;
END-ISO-10303-21;
